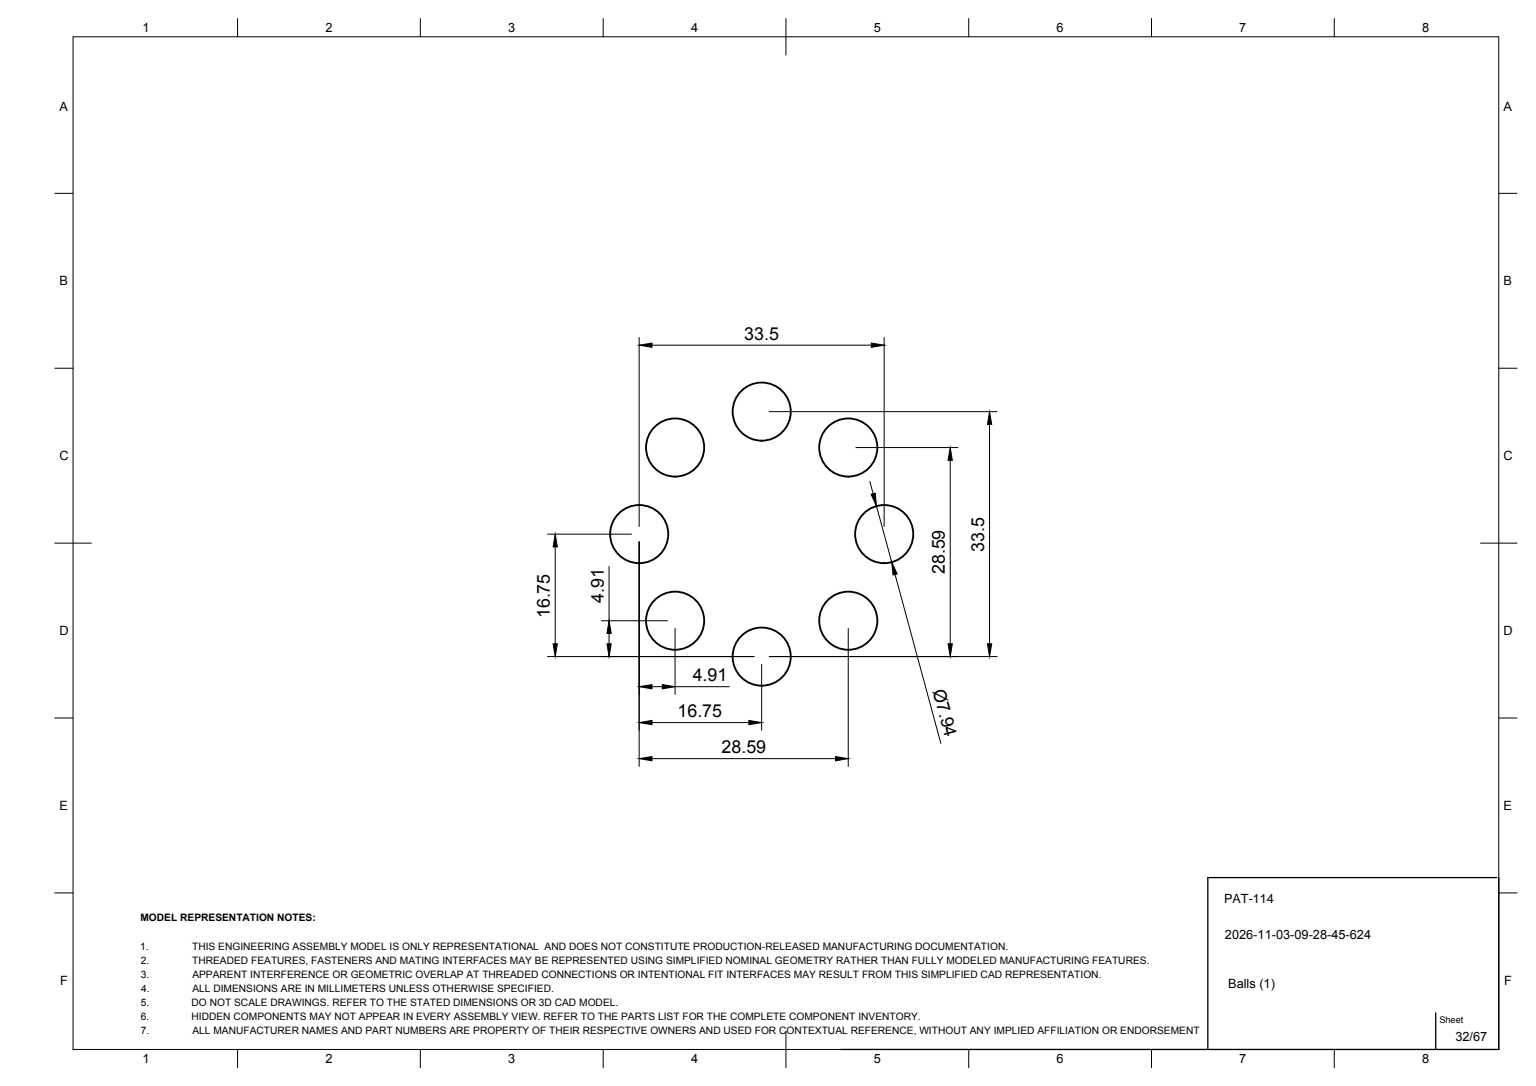
ISO-10303-21;
HEADER;
/* Generated by software containing ST-Developer
 * from STEP Tools, Inc. (www.steptools.com) 
 */

FILE_DESCRIPTION(
/* description */ ('Two-stage gear reducer in split housing'),
/* implementation_level */ '2;1');

FILE_NAME(
/* name */ 'Balls (1).step',
/* time_stamp */ '2026-10-28T03:22:31-07:00',
/* author */ (''),
/* organization */ (''),
/* preprocessor_version */ 'ST-DEVELOPER v20.2',
/* originating_system */ 'Autodesk Translation Framework v15.17.0.0',
/* authorisation */ '');

FILE_SCHEMA (('AUTOMOTIVE_DESIGN { 1 0 10303 214 3 1 1 }'));
ENDSEC;

DATA;
#10=MECHANICAL_DESIGN_GEOMETRIC_PRESENTATION_REPRESENTATION('',(#1265,#1266,#1267,#1268,#1269,#1270,#1271,#1272),#73366);
#1081=SPHERICAL_SURFACE('',#17586,0.3969);
#1082=SPHERICAL_SURFACE('',#17588,0.3969);
#1083=SPHERICAL_SURFACE('',#17590,0.3969);
#1084=SPHERICAL_SURFACE('',#17592,0.3969);
#1085=SPHERICAL_SURFACE('',#17594,0.3969);
#1086=SPHERICAL_SURFACE('',#17596,0.3969);
#1087=SPHERICAL_SURFACE('',#17598,0.3969);
#1088=SPHERICAL_SURFACE('',#17600,0.3969);
#1146=SHAPE_REPRESENTATION_RELATIONSHIP('SRR','None',#73635,#1202);
#1202=ADVANCED_BREP_SHAPE_REPRESENTATION('',(#1335,#1336,#1337,#1338,#1339,
#1340,#1341,#1342),#73331);
#1265=STYLED_ITEM('',(#73988),#1335);
#1266=STYLED_ITEM('',(#73988),#1336);
#1267=STYLED_ITEM('',(#73988),#1337);
#1268=STYLED_ITEM('',(#73988),#1338);
#1269=STYLED_ITEM('',(#73988),#1339);
#1270=STYLED_ITEM('',(#73988),#1340);
#1271=STYLED_ITEM('',(#73988),#1341);
#1272=STYLED_ITEM('',(#73988),#1342);
#1335=MANIFOLD_SOLID_BREP('Body1',#16154);
#1336=MANIFOLD_SOLID_BREP('Body2',#16155);
#1337=MANIFOLD_SOLID_BREP('Body3',#16156);
#1338=MANIFOLD_SOLID_BREP('Body4',#16157);
#1339=MANIFOLD_SOLID_BREP('Body5',#16158);
#1340=MANIFOLD_SOLID_BREP('Body6',#16159);
#1341=MANIFOLD_SOLID_BREP('Body7',#16160);
#1342=MANIFOLD_SOLID_BREP('Body8',#16161);
#2364=FACE_OUTER_BOUND('',#3435,.T.);
#2365=FACE_OUTER_BOUND('',#3436,.T.);
#2366=FACE_OUTER_BOUND('',#3437,.T.);
#2367=FACE_OUTER_BOUND('',#3438,.T.);
#2368=FACE_OUTER_BOUND('',#3439,.T.);
#2369=FACE_OUTER_BOUND('',#3440,.T.);
#2370=FACE_OUTER_BOUND('',#3441,.T.);
#2371=FACE_OUTER_BOUND('',#3442,.T.);
#3435=EDGE_LOOP('',(#12077,#12078));
#3436=EDGE_LOOP('',(#12079,#12080));
#3437=EDGE_LOOP('',(#12081,#12082));
#3438=EDGE_LOOP('',(#12083,#12084));
#3439=EDGE_LOOP('',(#12085,#12086));
#3440=EDGE_LOOP('',(#12087,#12088));
#3441=EDGE_LOOP('',(#12089,#12090));
#3442=EDGE_LOOP('',(#12091,#12092));
#6482=CIRCLE('',#17587,0.3969);
#6483=CIRCLE('',#17589,0.3969);
#6484=CIRCLE('',#17591,0.3969);
#6485=CIRCLE('',#17593,0.3969);
#6486=CIRCLE('',#17595,0.3969);
#6487=CIRCLE('',#17597,0.3969);
#6488=CIRCLE('',#17599,0.3969);
#6489=CIRCLE('',#17601,0.3969);
#7353=VERTEX_POINT('',#24779);
#7354=VERTEX_POINT('',#24780);
#7355=VERTEX_POINT('',#24783);
#7356=VERTEX_POINT('',#24784);
#7357=VERTEX_POINT('',#24787);
#7358=VERTEX_POINT('',#24788);
#7359=VERTEX_POINT('',#24791);
#7360=VERTEX_POINT('',#24792);
#7361=VERTEX_POINT('',#24795);
#7362=VERTEX_POINT('',#24796);
#7363=VERTEX_POINT('',#24799);
#7364=VERTEX_POINT('',#24800);
#7365=VERTEX_POINT('',#24803);
#7366=VERTEX_POINT('',#24804);
#7367=VERTEX_POINT('',#24807);
#7368=VERTEX_POINT('',#24808);
#9092=EDGE_CURVE('',#7353,#7354,#6482,.T.);
#9093=EDGE_CURVE('',#7355,#7356,#6483,.T.);
#9094=EDGE_CURVE('',#7357,#7358,#6484,.T.);
#9095=EDGE_CURVE('',#7359,#7360,#6485,.T.);
#9096=EDGE_CURVE('',#7361,#7362,#6486,.T.);
#9097=EDGE_CURVE('',#7363,#7364,#6487,.T.);
#9098=EDGE_CURVE('',#7365,#7366,#6488,.T.);
#9099=EDGE_CURVE('',#7367,#7368,#6489,.T.);
#12077=ORIENTED_EDGE('',*,*,#9092,.T.);
#12078=ORIENTED_EDGE('',*,*,#9092,.F.);
#12079=ORIENTED_EDGE('',*,*,#9093,.T.);
#12080=ORIENTED_EDGE('',*,*,#9093,.F.);
#12081=ORIENTED_EDGE('',*,*,#9094,.T.);
#12082=ORIENTED_EDGE('',*,*,#9094,.F.);
#12083=ORIENTED_EDGE('',*,*,#9095,.T.);
#12084=ORIENTED_EDGE('',*,*,#9095,.F.);
#12085=ORIENTED_EDGE('',*,*,#9096,.T.);
#12086=ORIENTED_EDGE('',*,*,#9096,.F.);
#12087=ORIENTED_EDGE('',*,*,#9097,.T.);
#12088=ORIENTED_EDGE('',*,*,#9097,.F.);
#12089=ORIENTED_EDGE('',*,*,#9098,.T.);
#12090=ORIENTED_EDGE('',*,*,#9098,.F.);
#12091=ORIENTED_EDGE('',*,*,#9099,.T.);
#12092=ORIENTED_EDGE('',*,*,#9099,.F.);
#15571=ADVANCED_FACE('',(#2364),#1081,.T.);
#15572=ADVANCED_FACE('',(#2365),#1082,.T.);
#15573=ADVANCED_FACE('',(#2366),#1083,.T.);
#15574=ADVANCED_FACE('',(#2367),#1084,.T.);
#15575=ADVANCED_FACE('',(#2368),#1085,.T.);
#15576=ADVANCED_FACE('',(#2369),#1086,.T.);
#15577=ADVANCED_FACE('',(#2370),#1087,.T.);
#15578=ADVANCED_FACE('',(#2371),#1088,.T.);
#16154=CLOSED_SHELL('',(#15571));
#16155=CLOSED_SHELL('',(#15572));
#16156=CLOSED_SHELL('',(#15573));
#16157=CLOSED_SHELL('',(#15574));
#16158=CLOSED_SHELL('',(#15575));
#16159=CLOSED_SHELL('',(#15576));
#16160=CLOSED_SHELL('',(#15577));
#16161=CLOSED_SHELL('',(#15578));
#17585=AXIS2_PLACEMENT_3D('',#24777,#20397,#20398);
#17586=AXIS2_PLACEMENT_3D('',#24778,#20399,#20400);
#17587=AXIS2_PLACEMENT_3D('',#24781,#20401,#20402);
#17588=AXIS2_PLACEMENT_3D('',#24782,#20403,#20404);
#17589=AXIS2_PLACEMENT_3D('',#24785,#20405,#20406);
#17590=AXIS2_PLACEMENT_3D('',#24786,#20407,#20408);
#17591=AXIS2_PLACEMENT_3D('',#24789,#20409,#20410);
#17592=AXIS2_PLACEMENT_3D('',#24790,#20411,#20412);
#17593=AXIS2_PLACEMENT_3D('',#24793,#20413,#20414);
#17594=AXIS2_PLACEMENT_3D('',#24794,#20415,#20416);
#17595=AXIS2_PLACEMENT_3D('',#24797,#20417,#20418);
#17596=AXIS2_PLACEMENT_3D('',#24798,#20419,#20420);
#17597=AXIS2_PLACEMENT_3D('',#24801,#20421,#20422);
#17598=AXIS2_PLACEMENT_3D('',#24802,#20423,#20424);
#17599=AXIS2_PLACEMENT_3D('',#24805,#20425,#20426);
#17600=AXIS2_PLACEMENT_3D('',#24806,#20427,#20428);
#17601=AXIS2_PLACEMENT_3D('',#24809,#20429,#20430);
#20397=DIRECTION('axis',(0.,0.,1.));
#20398=DIRECTION('refdir',(1.,0.,0.));
#20399=DIRECTION('center_axis',(0.,0.,1.));
#20400=DIRECTION('ref_axis',(1.,0.,0.));
#20401=DIRECTION('center_axis',(1.22464679914735E-16,-1.,0.));
#20402=DIRECTION('ref_axis',(-1.,-1.22464679914735E-16,0.));
#20403=DIRECTION('center_axis',(0.707106781186548,0.,0.707106781186548));
#20404=DIRECTION('ref_axis',(0.707106781186548,0.,-0.707106781186548));
#20405=DIRECTION('center_axis',(8.65956056235493E-17,-1.,-8.65956056235493E-17));
#20406=DIRECTION('ref_axis',(-0.707106781186548,-1.22464679914735E-16,0.707106781186548));
#20407=DIRECTION('center_axis',(1.,0.,0.));
#20408=DIRECTION('ref_axis',(6.12323399573677E-17,0.,-1.));
#20409=DIRECTION('center_axis',(7.49879891330929E-33,-1.,-1.22464679914735E-16));
#20410=DIRECTION('ref_axis',(-6.12323399573677E-17,-1.22464679914735E-16,
1.));
#20411=DIRECTION('center_axis',(0.707106781186548,0.,-0.707106781186548));
#20412=DIRECTION('ref_axis',(-0.707106781186548,0.,-0.707106781186548));
#20413=DIRECTION('center_axis',(-8.65956056235493E-17,-1.,-8.65956056235493E-17));
#20414=DIRECTION('ref_axis',(0.707106781186548,-1.22464679914735E-16,0.707106781186548));
#20415=DIRECTION('center_axis',(0.,0.,-1.));
#20416=DIRECTION('ref_axis',(-1.,0.,-1.22464679914735E-16));
#20417=DIRECTION('center_axis',(-1.22464679914735E-16,-1.,-1.49975978266186E-32));
#20418=DIRECTION('ref_axis',(1.,-1.22464679914735E-16,1.22464679914735E-16));
#20419=DIRECTION('center_axis',(-0.707106781186548,0.,-0.707106781186548));
#20420=DIRECTION('ref_axis',(-0.707106781186548,0.,0.707106781186548));
#20421=DIRECTION('center_axis',(-8.65956056235493E-17,-1.,8.65956056235493E-17));
#20422=DIRECTION('ref_axis',(0.707106781186548,-1.22464679914735E-16,-0.707106781186548));
#20423=DIRECTION('center_axis',(-1.,0.,0.));
#20424=DIRECTION('ref_axis',(-1.83697019872103E-16,0.,1.));
#20425=DIRECTION('center_axis',(-2.24963967399279E-32,-1.,1.22464679914735E-16));
#20426=DIRECTION('ref_axis',(1.83697019872103E-16,-1.22464679914735E-16,
-1.));
#20427=DIRECTION('center_axis',(-0.707106781186548,0.,0.707106781186548));
#20428=DIRECTION('ref_axis',(0.707106781186548,0.,0.707106781186548));
#20429=DIRECTION('center_axis',(8.65956056235493E-17,-1.,8.65956056235494E-17));
#20430=DIRECTION('ref_axis',(-0.707106781186548,-1.22464679914735E-16,-0.707106781186548));
#24777=CARTESIAN_POINT('',(0.,0.,0.));
#24778=CARTESIAN_POINT('Origin',(1.675,0.,0.));
#24779=CARTESIAN_POINT('',(1.675,-2.97627328869245E-33,0.3969));
#24780=CARTESIAN_POINT('',(1.675,-2.97627328869245E-33,-0.3969));
#24781=CARTESIAN_POINT('Origin',(1.675,0.,0.));
#24782=CARTESIAN_POINT('Origin',(1.18440385848747,0.,-1.18440385848747));
#24783=CARTESIAN_POINT('',(1.46505453994041,3.1867025333467E-33,-0.903753177034526));
#24784=CARTESIAN_POINT('',(0.903753177034527,-9.13924911073161E-33,-1.46505453994041));
#24785=CARTESIAN_POINT('Origin',(1.18440385848747,0.,-1.18440385848747));
#24786=CARTESIAN_POINT('Origin',(1.02564169428591E-16,0.,-1.675));
#24787=CARTESIAN_POINT('',(0.3969,-2.97627328869246E-33,-1.675));
#24788=CARTESIAN_POINT('',(-0.3969,-2.97627328869245E-33,-1.675));
#24789=CARTESIAN_POINT('Origin',(1.02564169428591E-16,0.,-1.675));
#24790=CARTESIAN_POINT('Origin',(-1.18440385848747,0.,-1.18440385848747));
#24791=CARTESIAN_POINT('',(-0.903753177034526,3.1867025333467E-33,-1.46505453994041));
#24792=CARTESIAN_POINT('',(-1.46505453994041,-9.13924911073161E-33,-0.903753177034527));
#24793=CARTESIAN_POINT('Origin',(-1.18440385848747,0.,-1.18440385848747));
#24794=CARTESIAN_POINT('Origin',(-1.675,0.,-2.05128338857182E-16));
#24795=CARTESIAN_POINT('',(-1.675,-2.97627328869246E-33,-0.3969));
#24796=CARTESIAN_POINT('',(-1.675,-2.97627328869245E-33,0.3969));
#24797=CARTESIAN_POINT('Origin',(-1.675,0.,-2.05128338857182E-16));
#24798=CARTESIAN_POINT('Origin',(-1.18440385848747,0.,1.18440385848747));
#24799=CARTESIAN_POINT('',(-1.46505453994041,6.26819044436628E-33,0.903753177034526));
#24800=CARTESIAN_POINT('',(-0.903753177034527,-1.22207370217512E-32,1.46505453994041));
#24801=CARTESIAN_POINT('Origin',(-1.18440385848747,0.,1.18440385848747));
#24802=CARTESIAN_POINT('Origin',(-3.07692508285772E-16,0.,1.675));
#24803=CARTESIAN_POINT('',(-0.3969,-2.97627328869246E-33,1.675));
#24804=CARTESIAN_POINT('',(0.396899999999999,-2.97627328869245E-33,1.675));
#24805=CARTESIAN_POINT('Origin',(-3.07692508285772E-16,0.,1.675));
#24806=CARTESIAN_POINT('Origin',(1.18440385848747,0.,1.18440385848747));
#24807=CARTESIAN_POINT('',(0.903753177034526,9.34967835538585E-33,1.46505453994041));
#24808=CARTESIAN_POINT('',(1.46505453994041,-1.53022249327708E-32,0.903753177034527));
#24809=CARTESIAN_POINT('Origin',(1.18440385848747,0.,1.18440385848747));
#73267=UNCERTAINTY_MEASURE_WITH_UNIT(LENGTH_MEASURE(0.001),#73367,
'DISTANCE_ACCURACY_VALUE',
'Maximum model space distance between geometric entities at asserted c
onnectivities');
#73302=UNCERTAINTY_MEASURE_WITH_UNIT(LENGTH_MEASURE(0.001),#73367,
'DISTANCE_ACCURACY_VALUE',
'Maximum model space distance between geometric entities at asserted c
onnectivities');
#73331=(
GEOMETRIC_REPRESENTATION_CONTEXT(3)
GLOBAL_UNCERTAINTY_ASSIGNED_CONTEXT((#73267))
GLOBAL_UNIT_ASSIGNED_CONTEXT((#73367,#73369,#73370))
REPRESENTATION_CONTEXT('','3D')
);
#73366=(
GEOMETRIC_REPRESENTATION_CONTEXT(3)
GLOBAL_UNCERTAINTY_ASSIGNED_CONTEXT((#73302))
GLOBAL_UNIT_ASSIGNED_CONTEXT((#73367,#73369,#73370))
REPRESENTATION_CONTEXT('','3D')
);
#73367=(
LENGTH_UNIT()
NAMED_UNIT(*)
SI_UNIT(.CENTI.,.METRE.)
);
#73369=(
NAMED_UNIT(*)
PLANE_ANGLE_UNIT()
SI_UNIT($,.RADIAN.)
);
#73370=(
NAMED_UNIT(*)
SI_UNIT($,.STERADIAN.)
SOLID_ANGLE_UNIT()
);
#73399=SHAPE_DEFINITION_REPRESENTATION(#73467,#73635);
#73467=PRODUCT_DEFINITION_SHAPE('',$,#73699);
#73635=SHAPE_REPRESENTATION('',(#17585),#73331);
#73670=PRODUCT_DEFINITION_CONTEXT('part definition',#73861,'design');
#73699=PRODUCT_DEFINITION('Balls (1)','Balls (1)',#73762,#73670);
#73762=PRODUCT_DEFINITION_FORMATION('',$,#73891);
#73861=APPLICATION_CONTEXT(
'Core Data for Automotive Mechanical Design Process');
#73862=PRODUCT_CONTEXT('part definition',#73861,'mechanical');
#73891=PRODUCT('Balls (1)','Balls (1)','Balls (1)',(#73862));
#73982=COLOUR_RGB('Grey',0.48,0.52,0.57);
#73983=FILL_AREA_STYLE_COLOUR('',#73982);
#73984=FILL_AREA_STYLE('',(#73983));
#73985=SURFACE_STYLE_FILL_AREA(#73984);
#73986=SURFACE_SIDE_STYLE('',(#73985));
#73987=SURFACE_STYLE_USAGE(.BOTH.,#73986);
#73988=PRESENTATION_STYLE_ASSIGNMENT((#73987));
ENDSEC;
END-ISO-10303-21;
